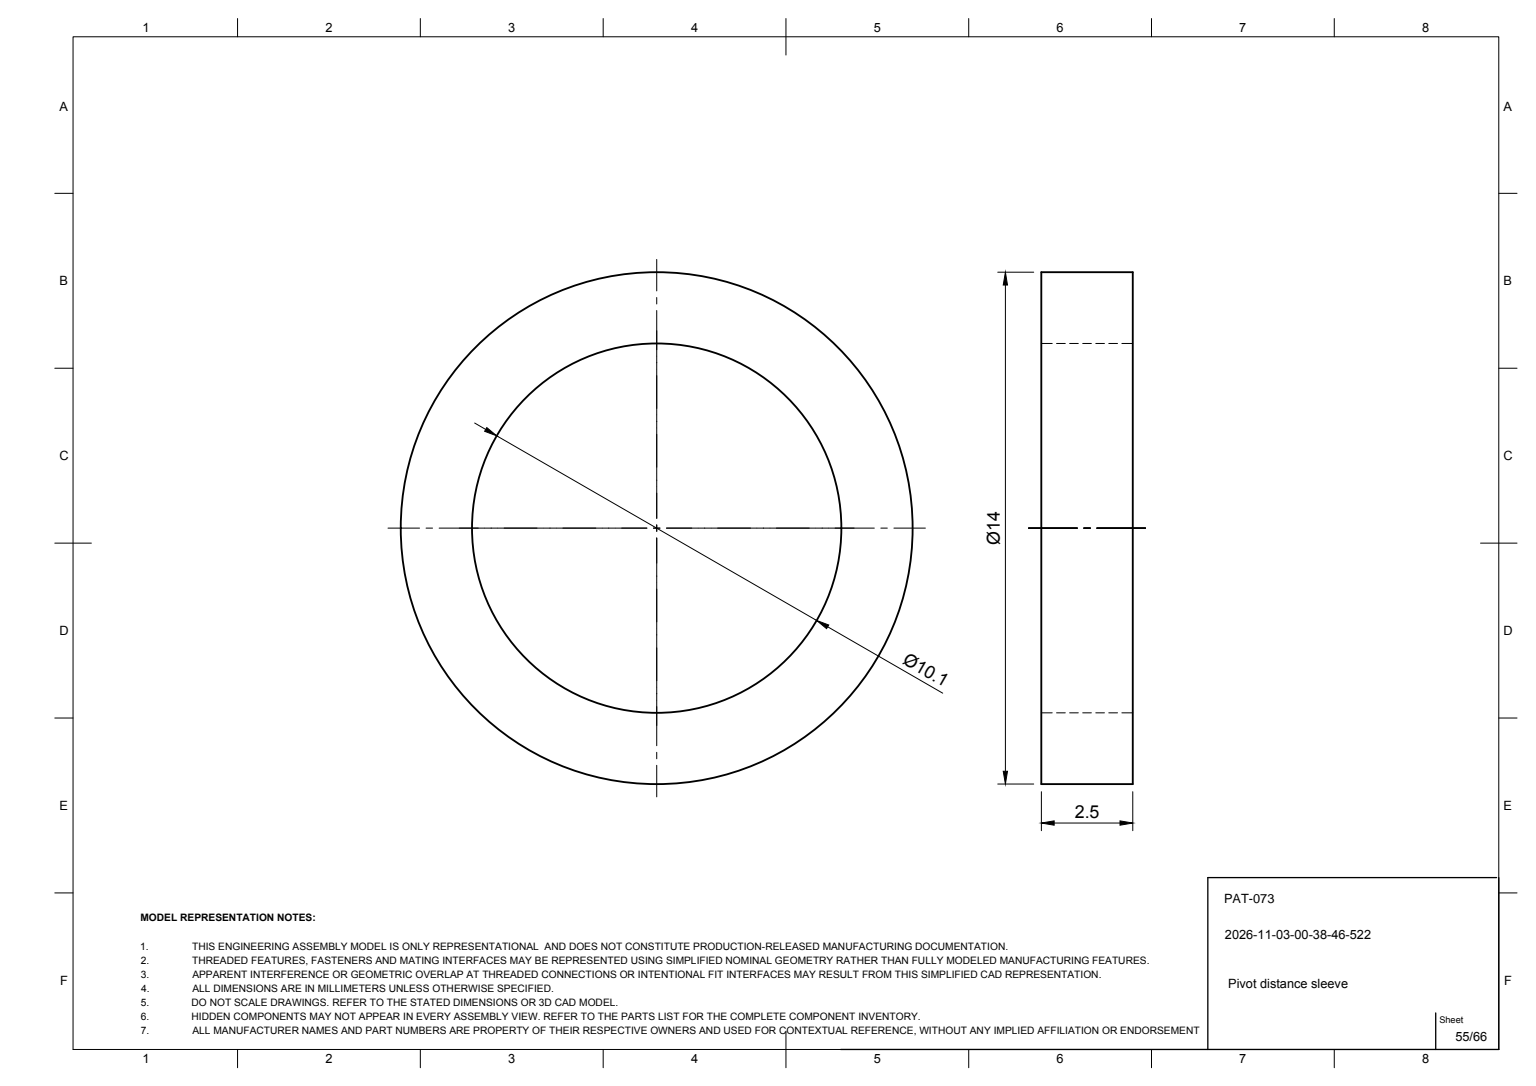
ISO-10303-21;
HEADER;
/* Generated by software containing ST-Developer
 * from STEP Tools, Inc. (www.steptools.com) 
 */

FILE_DESCRIPTION(
/* description */ ('Manual piston pump'),
/* implementation_level */ '2;1');

FILE_NAME(
/* name */ 'Pivot distance sleeve.step',
/* time_stamp */ '2026-11-02T16:54:23-08:00',
/* author */ (''),
/* organization */ (''),
/* preprocessor_version */ 'ST-DEVELOPER v20.2',
/* originating_system */ 'Autodesk Translation Framework v15.17.0.0',
/* authorisation */ '');

FILE_SCHEMA (('AUTOMOTIVE_DESIGN { 1 0 10303 214 3 1 1 }'));
ENDSEC;

DATA;
#10=MECHANICAL_DESIGN_GEOMETRIC_PRESENTATION_REPRESENTATION('',(#745),#19043);
#611=SHAPE_REPRESENTATION_RELATIONSHIP('SRR','None',#19361,#674);
#674=ADVANCED_BREP_SHAPE_REPRESENTATION('',(#813),#19028);
#745=STYLED_ITEM('',(#19664),#813);
#813=MANIFOLD_SOLID_BREP('Body1',#9533);
#1020=FACE_BOUND('',#2537,.T.);
#1021=FACE_BOUND('',#2539,.T.);
#1257=CYLINDRICAL_SURFACE('',#11274,0.505000000000001);
#1258=CYLINDRICAL_SURFACE('',#11277,0.699999999999999);
#1766=FACE_OUTER_BOUND('',#2534,.T.);
#1767=FACE_OUTER_BOUND('',#2535,.T.);
#1768=FACE_OUTER_BOUND('',#2536,.T.);
#1769=FACE_OUTER_BOUND('',#2538,.T.);
#2534=EDGE_LOOP('',(#8173,#8174,#8175,#8176));
#2535=EDGE_LOOP('',(#8177,#8178,#8179,#8180));
#2536=EDGE_LOOP('',(#8181));
#2537=EDGE_LOOP('',(#8182));
#2538=EDGE_LOOP('',(#8183));
#2539=EDGE_LOOP('',(#8184));
#3072=CIRCLE('',#11275,0.505000000000001);
#3073=CIRCLE('',#11276,0.505000000000001);
#3074=CIRCLE('',#11278,0.699999999999999);
#3075=CIRCLE('',#11279,0.699999999999999);
#3640=LINE('',#18319,#4244);
#3641=LINE('',#18325,#4245);
#4244=VECTOR('',#14054,0.505000000000001);
#4245=VECTOR('',#14061,0.699999999999999);
#4992=VERTEX_POINT('',#18316);
#4993=VERTEX_POINT('',#18318);
#4994=VERTEX_POINT('',#18322);
#4995=VERTEX_POINT('',#18324);
#6073=EDGE_CURVE('',#4992,#4992,#3072,.T.);
#6074=EDGE_CURVE('',#4992,#4993,#3640,.T.);
#6075=EDGE_CURVE('',#4993,#4993,#3073,.T.);
#6076=EDGE_CURVE('',#4994,#4994,#3074,.T.);
#6077=EDGE_CURVE('',#4994,#4995,#3641,.T.);
#6078=EDGE_CURVE('',#4995,#4995,#3075,.T.);
#8173=ORIENTED_EDGE('',*,*,#6073,.F.);
#8174=ORIENTED_EDGE('',*,*,#6074,.T.);
#8175=ORIENTED_EDGE('',*,*,#6075,.T.);
#8176=ORIENTED_EDGE('',*,*,#6074,.F.);
#8177=ORIENTED_EDGE('',*,*,#6076,.F.);
#8178=ORIENTED_EDGE('',*,*,#6077,.T.);
#8179=ORIENTED_EDGE('',*,*,#6078,.T.);
#8180=ORIENTED_EDGE('',*,*,#6077,.F.);
#8181=ORIENTED_EDGE('',*,*,#6076,.T.);
#8182=ORIENTED_EDGE('',*,*,#6073,.T.);
#8183=ORIENTED_EDGE('',*,*,#6078,.F.);
#8184=ORIENTED_EDGE('',*,*,#6075,.F.);
#8836=PLANE('',#11280);
#8837=PLANE('',#11281);
#9371=ADVANCED_FACE('',(#1766),#1257,.F.);
#9372=ADVANCED_FACE('',(#1767),#1258,.T.);
#9373=ADVANCED_FACE('',(#1768,#1020),#8836,.T.);
#9374=ADVANCED_FACE('',(#1769,#1021),#8837,.F.);
#9533=CLOSED_SHELL('',(#9371,#9372,#9373,#9374));
#11273=AXIS2_PLACEMENT_3D('',#18314,#14048,#14049);
#11274=AXIS2_PLACEMENT_3D('',#18315,#14050,#14051);
#11275=AXIS2_PLACEMENT_3D('',#18317,#14052,#14053);
#11276=AXIS2_PLACEMENT_3D('',#18320,#14055,#14056);
#11277=AXIS2_PLACEMENT_3D('',#18321,#14057,#14058);
#11278=AXIS2_PLACEMENT_3D('',#18323,#14059,#14060);
#11279=AXIS2_PLACEMENT_3D('',#18326,#14062,#14063);
#11280=AXIS2_PLACEMENT_3D('',#18327,#14064,#14065);
#11281=AXIS2_PLACEMENT_3D('',#18328,#14066,#14067);
#14048=DIRECTION('axis',(0.,0.,1.));
#14049=DIRECTION('refdir',(1.,0.,0.));
#14050=DIRECTION('center_axis',(1.,0.,0.));
#14051=DIRECTION('ref_axis',(0.,0.,-1.));
#14052=DIRECTION('center_axis',(-1.,0.,0.));
#14053=DIRECTION('ref_axis',(0.,0.,-1.));
#14054=DIRECTION('',(-1.,0.,0.));
#14055=DIRECTION('center_axis',(-1.,0.,0.));
#14056=DIRECTION('ref_axis',(0.,0.,-1.));
#14057=DIRECTION('center_axis',(1.,0.,0.));
#14058=DIRECTION('ref_axis',(0.,0.,-1.));
#14059=DIRECTION('center_axis',(1.,0.,0.));
#14060=DIRECTION('ref_axis',(0.,0.,-1.));
#14061=DIRECTION('',(-1.,0.,0.));
#14062=DIRECTION('center_axis',(1.,0.,0.));
#14063=DIRECTION('ref_axis',(0.,0.,-1.));
#14064=DIRECTION('center_axis',(1.,0.,0.));
#14065=DIRECTION('ref_axis',(0.,0.,-1.));
#14066=DIRECTION('center_axis',(1.,0.,0.));
#14067=DIRECTION('ref_axis',(0.,0.,-1.));
#18314=CARTESIAN_POINT('',(0.,0.,0.));
#18315=CARTESIAN_POINT('Origin',(-3.2,-4.,10.));
#18316=CARTESIAN_POINT('',(-2.95,-4.,10.505));
#18317=CARTESIAN_POINT('Origin',(-2.95,-4.,10.));
#18318=CARTESIAN_POINT('',(-3.2,-4.,10.505));
#18319=CARTESIAN_POINT('',(-3.2,-4.,10.505));
#18320=CARTESIAN_POINT('Origin',(-3.2,-4.,10.));
#18321=CARTESIAN_POINT('Origin',(-3.2,-4.,10.));
#18322=CARTESIAN_POINT('',(-2.95,-4.,10.7));
#18323=CARTESIAN_POINT('Origin',(-2.95,-4.,10.));
#18324=CARTESIAN_POINT('',(-3.2,-4.,10.7));
#18325=CARTESIAN_POINT('',(-3.2,-4.,10.7));
#18326=CARTESIAN_POINT('Origin',(-3.2,-4.,10.));
#18327=CARTESIAN_POINT('Origin',(-2.95,-4.,10.));
#18328=CARTESIAN_POINT('Origin',(-3.2,-4.,10.));
#18957=UNCERTAINTY_MEASURE_WITH_UNIT(LENGTH_MEASURE(0.001),#19044,
'DISTANCE_ACCURACY_VALUE',
'Maximum model space distance between geometric entities at asserted c
onnectivities');
#18972=UNCERTAINTY_MEASURE_WITH_UNIT(LENGTH_MEASURE(0.001),#19044,
'DISTANCE_ACCURACY_VALUE',
'Maximum model space distance between geometric entities at asserted c
onnectivities');
#19028=(
GEOMETRIC_REPRESENTATION_CONTEXT(3)
GLOBAL_UNCERTAINTY_ASSIGNED_CONTEXT((#18957))
GLOBAL_UNIT_ASSIGNED_CONTEXT((#19044,#19046,#19047))
REPRESENTATION_CONTEXT('','3D')
);
#19043=(
GEOMETRIC_REPRESENTATION_CONTEXT(3)
GLOBAL_UNCERTAINTY_ASSIGNED_CONTEXT((#18972))
GLOBAL_UNIT_ASSIGNED_CONTEXT((#19044,#19046,#19047))
REPRESENTATION_CONTEXT('','3D')
);
#19044=(
LENGTH_UNIT()
NAMED_UNIT(*)
SI_UNIT(.CENTI.,.METRE.)
);
#19046=(
NAMED_UNIT(*)
PLANE_ANGLE_UNIT()
SI_UNIT($,.RADIAN.)
);
#19047=(
NAMED_UNIT(*)
SI_UNIT($,.STERADIAN.)
SOLID_ANGLE_UNIT()
);
#19103=SHAPE_DEFINITION_REPRESENTATION(#19260,#19361);
#19260=PRODUCT_DEFINITION_SHAPE('',$,#19432);
#19361=SHAPE_REPRESENTATION('',(#11273),#19028);
#19376=PRODUCT_DEFINITION_CONTEXT('part definition',#19588,'design');
#19432=PRODUCT_DEFINITION('2026-11-03-00-38-46-522',
'Pivot distance sleeve',#19502,#19376);
#19502=PRODUCT_DEFINITION_FORMATION('',$,#19645);
#19588=APPLICATION_CONTEXT(
'Core Data for Automotive Mechanical Design Process');
#19589=PRODUCT_CONTEXT('part definition',#19588,'mechanical');
#19645=PRODUCT('2026-11-03-00-38-46-522','Pivot distance sleeve',
'Pivot distance sleeve',(#19589));
#19664=PRESENTATION_STYLE_ASSIGNMENT((#19670));
#19670=SURFACE_STYLE_USAGE(.BOTH.,#19676);
#19676=SURFACE_SIDE_STYLE('',(#19682));
#19682=SURFACE_STYLE_FILL_AREA(#19688);
#19688=FILL_AREA_STYLE('CAD Library Painted - Steel gray',(#19694));
#19694=FILL_AREA_STYLE_COLOUR('CAD Library Painted - Steel gray',#19700);
#19700=COLOUR_RGB('CAD Library Painted - Steel gray',0.592156862745098,
0.631372549019608,0.67843137254902);
ENDSEC;
END-ISO-10303-21;
